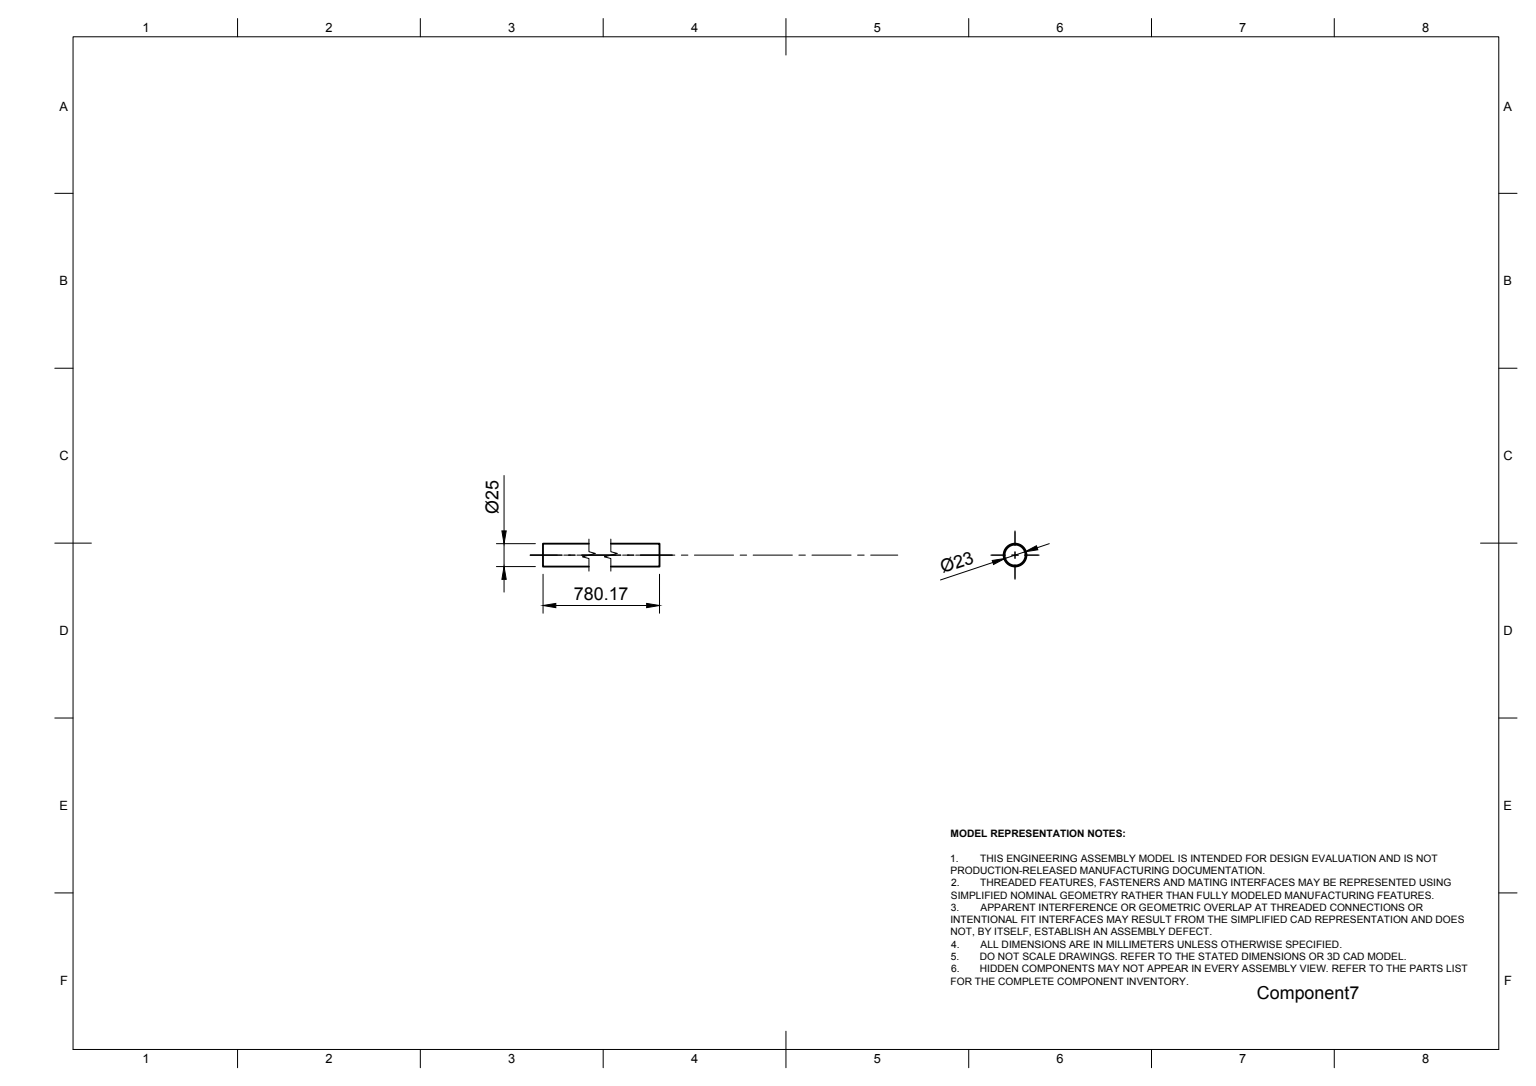
ISO-10303-21;
HEADER;
/* Generated by software containing ST-Developer
 * from STEP Tools, Inc. (www.steptools.com) 
 */

FILE_DESCRIPTION(
/* description */ ('STEP AP214'),
/* implementation_level */ '2;1');

FILE_NAME(
/* name */ 'Component7.step',
/* time_stamp */ '2026-10-06T11:02:40-07:00',
/* author */ (''),
/* organization */ (''),
/* preprocessor_version */ 'ST-DEVELOPER v20.2',
/* originating_system */ 'Autodesk Translation Framework v15.15.0.0',
/* authorisation */ '');

FILE_SCHEMA (('AUTOMOTIVE_DESIGN { 1 0 10303 214 3 1 1 }'));
ENDSEC;

DATA;
#10=MECHANICAL_DESIGN_GEOMETRIC_PRESENTATION_REPRESENTATION('',(#2942),#130910);
#731=FACE_BOUND('',#15335,.T.);
#2926=SHAPE_REPRESENTATION_RELATIONSHIP('SRR','None',#130948,#2934);
#2934=ADVANCED_BREP_SHAPE_REPRESENTATION('',(#2948),#130908);
#2942=STYLED_ITEM('',(#130991),#2948);
#2948=MANIFOLD_SOLID_BREP('Body1',#45458);
#3643=PLANE('',#48899);
#3644=PLANE('',#48900);
#3645=PLANE('',#48901);
#5300=LINE('',#106580,#7074);
#5301=LINE('',#106586,#7075);
#7074=VECTOR('',#59281,11.5);
#7075=VECTOR('',#59288,12.5);
#8682=CYLINDRICAL_SURFACE('',#48893,11.5);
#8683=CYLINDRICAL_SURFACE('',#48896,12.5);
#11282=FACE_OUTER_BOUND('',#15331,.T.);
#11283=FACE_OUTER_BOUND('',#15332,.T.);
#11284=FACE_OUTER_BOUND('',#15333,.T.);
#11285=FACE_OUTER_BOUND('',#15334,.T.);
#11286=FACE_OUTER_BOUND('',#15336,.T.);
#15331=EDGE_LOOP('',(#36808,#36809,#36810,#36811));
#15332=EDGE_LOOP('',(#36812,#36813,#36814,#36815));
#15333=EDGE_LOOP('',(#36816));
#15334=EDGE_LOOP('',(#36817));
#15335=EDGE_LOOP('',(#36818));
#15336=EDGE_LOOP('',(#36819));
#19400=CIRCLE('',#48894,11.5);
#19401=CIRCLE('',#48895,11.5);
#19402=CIRCLE('',#48897,12.5);
#19403=CIRCLE('',#48898,12.5);
#22730=VERTEX_POINT('',#106577);
#22731=VERTEX_POINT('',#106579);
#22732=VERTEX_POINT('',#106583);
#22733=VERTEX_POINT('',#106585);
#27748=EDGE_CURVE('',#22730,#22730,#19400,.T.);
#27749=EDGE_CURVE('',#22730,#22731,#5300,.T.);
#27750=EDGE_CURVE('',#22731,#22731,#19401,.T.);
#27751=EDGE_CURVE('',#22732,#22732,#19402,.T.);
#27752=EDGE_CURVE('',#22732,#22733,#5301,.T.);
#27753=EDGE_CURVE('',#22733,#22733,#19403,.T.);
#36808=ORIENTED_EDGE('',*,*,#27748,.F.);
#36809=ORIENTED_EDGE('',*,*,#27749,.T.);
#36810=ORIENTED_EDGE('',*,*,#27750,.T.);
#36811=ORIENTED_EDGE('',*,*,#27749,.F.);
#36812=ORIENTED_EDGE('',*,*,#27751,.F.);
#36813=ORIENTED_EDGE('',*,*,#27752,.T.);
#36814=ORIENTED_EDGE('',*,*,#27753,.T.);
#36815=ORIENTED_EDGE('',*,*,#27752,.F.);
#36816=ORIENTED_EDGE('',*,*,#27753,.F.);
#36817=ORIENTED_EDGE('',*,*,#27751,.T.);
#36818=ORIENTED_EDGE('',*,*,#27750,.F.);
#36819=ORIENTED_EDGE('',*,*,#27748,.T.);
#43862=ADVANCED_FACE('',(#11282),#8682,.F.);
#43863=ADVANCED_FACE('',(#11283),#8683,.T.);
#43864=ADVANCED_FACE('',(#11284),#3643,.F.);
#43865=ADVANCED_FACE('',(#11285,#731),#3644,.T.);
#43866=ADVANCED_FACE('',(#11286),#3645,.T.);
#45458=CLOSED_SHELL('',(#43862,#43863,#43864,#43865,#43866));
#48892=AXIS2_PLACEMENT_3D('',#106575,#59275,#59276);
#48893=AXIS2_PLACEMENT_3D('',#106576,#59277,#59278);
#48894=AXIS2_PLACEMENT_3D('',#106578,#59279,#59280);
#48895=AXIS2_PLACEMENT_3D('',#106581,#59282,#59283);
#48896=AXIS2_PLACEMENT_3D('',#106582,#59284,#59285);
#48897=AXIS2_PLACEMENT_3D('',#106584,#59286,#59287);
#48898=AXIS2_PLACEMENT_3D('',#106587,#59289,#59290);
#48899=AXIS2_PLACEMENT_3D('',#106588,#59291,#59292);
#48900=AXIS2_PLACEMENT_3D('',#106589,#59293,#59294);
#48901=AXIS2_PLACEMENT_3D('',#106590,#59295,#59296);
#59275=DIRECTION('axis',(0.,0.,1.));
#59276=DIRECTION('refdir',(1.,0.,0.));
#59277=DIRECTION('center_axis',(0.,1.,0.));
#59278=DIRECTION('ref_axis',(0.,0.,1.));
#59279=DIRECTION('center_axis',(0.,1.,0.));
#59280=DIRECTION('ref_axis',(0.,0.,1.));
#59281=DIRECTION('',(0.,1.,0.));
#59282=DIRECTION('center_axis',(0.,1.,0.));
#59283=DIRECTION('ref_axis',(0.,0.,1.));
#59284=DIRECTION('center_axis',(0.,1.,0.));
#59285=DIRECTION('ref_axis',(0.,0.,1.));
#59286=DIRECTION('center_axis',(0.,1.,0.));
#59287=DIRECTION('ref_axis',(0.,0.,1.));
#59288=DIRECTION('',(0.,-1.,0.));
#59289=DIRECTION('center_axis',(0.,1.,0.));
#59290=DIRECTION('ref_axis',(0.,0.,1.));
#59291=DIRECTION('center_axis',(0.,1.,0.));
#59292=DIRECTION('ref_axis',(0.,0.,1.));
#59293=DIRECTION('center_axis',(0.,1.,0.));
#59294=DIRECTION('ref_axis',(0.,0.,1.));
#59295=DIRECTION('center_axis',(0.,1.,0.));
#59296=DIRECTION('ref_axis',(0.,0.,1.));
#106575=CARTESIAN_POINT('',(0.,0.,0.));
#106576=CARTESIAN_POINT('Origin',(0.,59.,64.2994740882088));
#106577=CARTESIAN_POINT('',(-1.40834381901946E-15,60.,52.7994740882088));
#106578=CARTESIAN_POINT('Origin',(0.,60.,64.2994740882088));
#106579=CARTESIAN_POINT('',(-1.40834381901946E-15,829.165008980169,52.7994740882088));
#106580=CARTESIAN_POINT('',(-1.40834381901946E-15,59.,52.7994740882088));
#106581=CARTESIAN_POINT('Origin',(0.,829.165008980169,64.2994740882095));
#106582=CARTESIAN_POINT('Origin',(0.,59.,64.2994740882088));
#106583=CARTESIAN_POINT('',(-1.53080849893419E-15,829.165008980169,51.7994740882088));
#106584=CARTESIAN_POINT('Origin',(0.,829.165008980169,64.2994740882088));
#106585=CARTESIAN_POINT('',(-1.53080849893419E-15,49.,51.7994740882088));
#106586=CARTESIAN_POINT('',(-1.53080849893419E-15,59.,51.7994740882088));
#106587=CARTESIAN_POINT('Origin',(0.,49.,64.2994740882088));
#106588=CARTESIAN_POINT('Origin',(0.,49.,64.2994740882088));
#106589=CARTESIAN_POINT('Origin',(0.,829.165008980169,76.7994740882088));
#106590=CARTESIAN_POINT('Origin',(0.,60.,64.2994740882088));
#130898=UNCERTAINTY_MEASURE_WITH_UNIT(LENGTH_MEASURE(0.01),#130911,
'DISTANCE_ACCURACY_VALUE',
'Maximum model space distance between geometric entities at asserted c
onnectivities');
#130900=UNCERTAINTY_MEASURE_WITH_UNIT(LENGTH_MEASURE(0.01),#130911,
'DISTANCE_ACCURACY_VALUE',
'Maximum model space distance between geometric entities at asserted c
onnectivities');
#130908=(
GEOMETRIC_REPRESENTATION_CONTEXT(3)
GLOBAL_UNCERTAINTY_ASSIGNED_CONTEXT((#130898))
GLOBAL_UNIT_ASSIGNED_CONTEXT((#130911,#130913,#130914))
REPRESENTATION_CONTEXT('','3D')
);
#130910=(
GEOMETRIC_REPRESENTATION_CONTEXT(3)
GLOBAL_UNCERTAINTY_ASSIGNED_CONTEXT((#130900))
GLOBAL_UNIT_ASSIGNED_CONTEXT((#130911,#130913,#130914))
REPRESENTATION_CONTEXT('','3D')
);
#130911=(
LENGTH_UNIT()
NAMED_UNIT(*)
SI_UNIT(.MILLI.,.METRE.)
);
#130913=(
NAMED_UNIT(*)
PLANE_ANGLE_UNIT()
SI_UNIT($,.RADIAN.)
);
#130914=(
NAMED_UNIT(*)
SI_UNIT($,.STERADIAN.)
SOLID_ANGLE_UNIT()
);
#130922=SHAPE_DEFINITION_REPRESENTATION(#130931,#130948);
#130931=PRODUCT_DEFINITION_SHAPE('',$,#130958);
#130948=SHAPE_REPRESENTATION('',(#48892),#130908);
#130950=PRODUCT_DEFINITION_CONTEXT('part definition',#130979,'design');
#130958=PRODUCT_DEFINITION('Component7','Component7',#130967,#130950);
#130967=PRODUCT_DEFINITION_FORMATION('',$,#130988);
#130979=APPLICATION_CONTEXT(
'Core Data for Automotive Mechanical Design Process');
#130980=PRODUCT_CONTEXT('part definition',#130979,'mechanical');
#130988=PRODUCT('Component7','Component7',$,(#130980));
#130991=PRESENTATION_STYLE_ASSIGNMENT((#130993));
#130993=SURFACE_STYLE_USAGE(.BOTH.,#130995);
#130995=SURFACE_SIDE_STYLE('',(#130997));
#130997=SURFACE_STYLE_FILL_AREA(#130999);
#130999=FILL_AREA_STYLE('Opaque(202,209,238)',(#131001));
#131001=FILL_AREA_STYLE_COLOUR('Opaque(202,209,238)',#131003);
#131003=COLOUR_RGB('Opaque(202,209,238)', 0.40784314, 0.44705882, 0.49803922);
ENDSEC;
END-ISO-10303-21;
